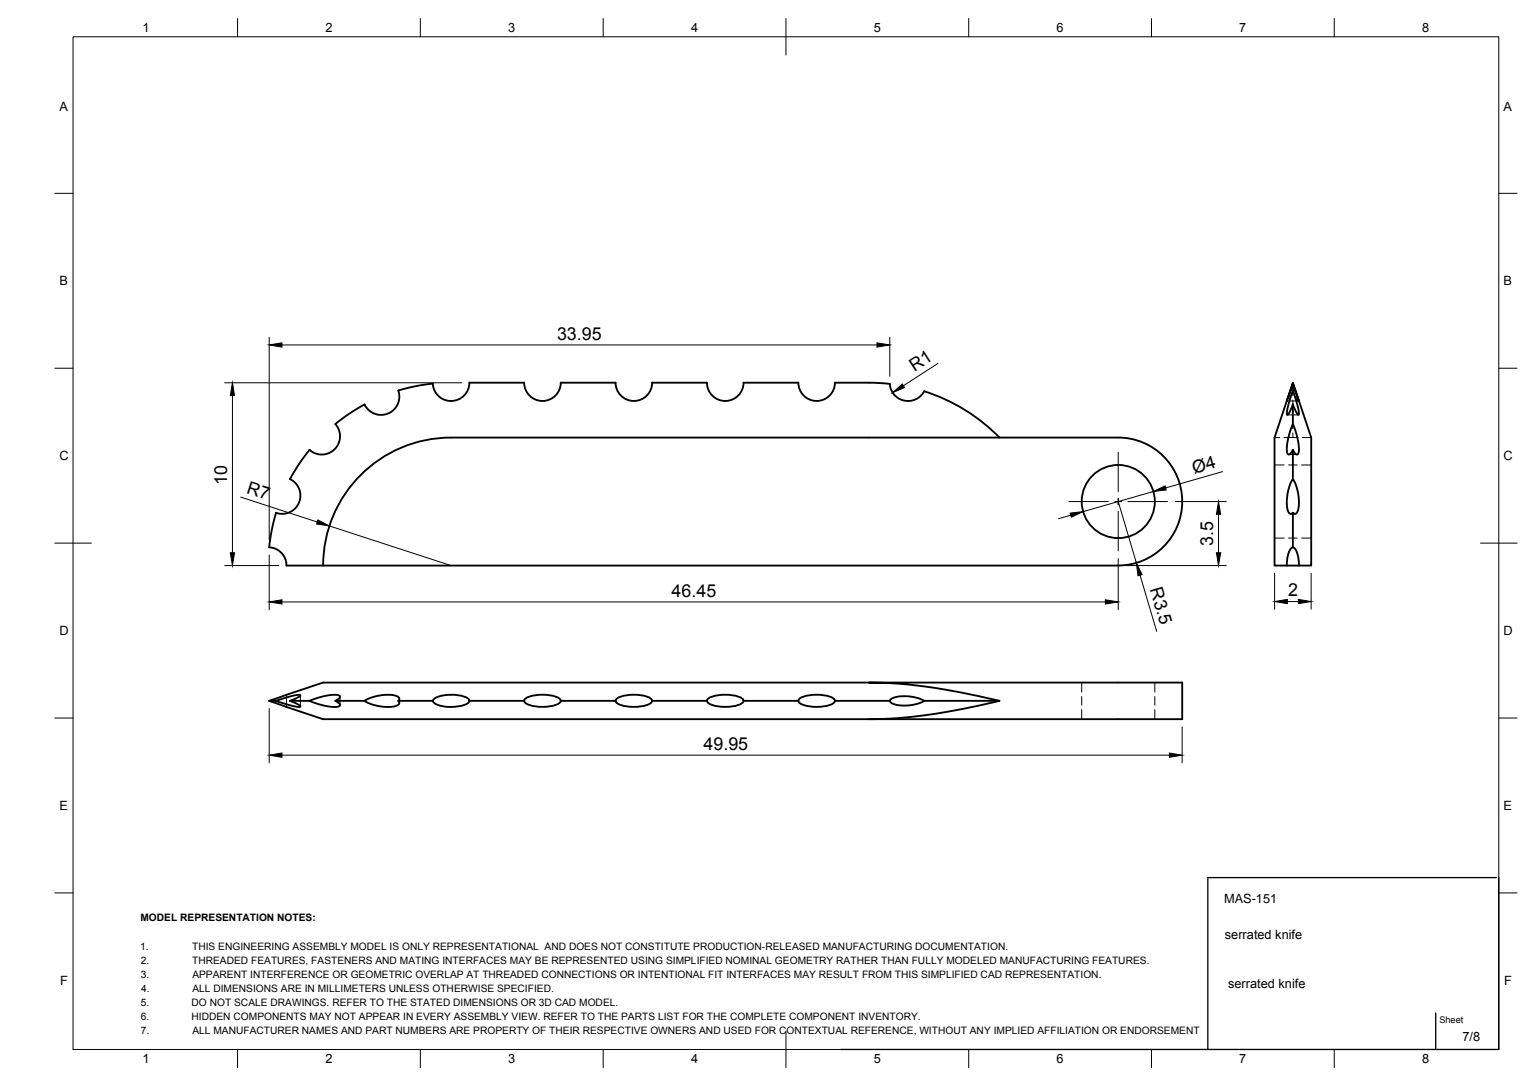
ISO-10303-21;
HEADER;
/* Generated by software containing ST-Developer
 * from STEP Tools, Inc. (www.steptools.com) 
 */

FILE_DESCRIPTION(
/* description */ ('STEP AP214'),
/* implementation_level */ '2;1');

FILE_NAME(
/* name */ 'serrated knife.step',
/* time_stamp */ '2026-11-04T19:14:12-08:00',
/* author */ (''),
/* organization */ (''),
/* preprocessor_version */ 'ST-DEVELOPER v20.2',
/* originating_system */ 'Autodesk Translation Framework v15.17.0.0',
/* authorisation */ '');

FILE_SCHEMA (('AUTOMOTIVE_DESIGN { 1 0 10303 214 3 1 1 }'));
ENDSEC;

DATA;
#10=MECHANICAL_DESIGN_GEOMETRIC_PRESENTATION_REPRESENTATION('',(#102),#5990);
#49=ELLIPSE('',#3546,1.05409255338808,0.99999999999868);
#50=ELLIPSE('',#3547,1.05409255338732,0.999999999998124);
#51=ELLIPSE('',#3549,1.05409255339022,1.00000000000065);
#52=ELLIPSE('',#3550,1.05409255338729,0.999999999997981);
#53=ELLIPSE('',#3552,1.05409255338844,0.99999999999902);
#54=ELLIPSE('',#3553,1.05409255338858,0.999999999999168);
#55=ELLIPSE('',#3555,1.05409255338794,0.999999999998691);
#56=ELLIPSE('',#3556,1.05409255338792,0.999999999998643);
#57=ELLIPSE('',#3558,1.05409255338783,0.999999999998475);
#58=ELLIPSE('',#3559,1.05409255338765,0.999999999998245);
#59=B_SPLINE_CURVE_WITH_KNOTS('',3,(#5264,#5265,#5266,#5267,#5268,#5269,
#5270,#5271,#5272,#5273,#5274,#5275,#5276,#5277,#5278,#5279,#5280,#5281),
 .UNSPECIFIED.,.F.,.F.,(4,2,2,2,2,2,2,2,4),(-0.601003528896593,-0.581975187755184,
-0.544665520692116,-0.509562261507989,-0.474459002323862,-0.439355743139737,
-0.404252483955611,-0.366942816892543,-0.347914475751133),.UNSPECIFIED.);
#60=B_SPLINE_CURVE_WITH_KNOTS('',3,(#5282,#5283,#5284,#5285,#5286,#5287,
#5288,#5289,#5290,#5291,#5292,#5293,#5294,#5295,#5296,#5297,#5298,#5299),
 .UNSPECIFIED.,.F.,.F.,(4,2,2,2,2,2,2,2,4),(-0.27137037906712,-0.252342037925712,
-0.215032370862644,-0.179929111678516,-0.144825852494388,-0.109722593310262,
-0.0746193341261349,-0.0373096670630674,-0.0182813259216579),
 .UNSPECIFIED.);
#61=B_SPLINE_CURVE_WITH_KNOTS('',3,(#5323,#5324,#5325,#5326,#5327,#5328,
#5329,#5330,#5331,#5332,#5333,#5334,#5335),.UNSPECIFIED.,.F.,.F.,(4,3,2,
2,2,4),(-0.00524378789543694,-6.24500451351651E-17,0.037252819941784,0.0745056398835681,
0.109553010570145,0.144600381256721),.UNSPECIFIED.);
#62=B_SPLINE_CURVE_WITH_KNOTS('',3,(#5340,#5341,#5342,#5343,#5344,#5345,
#5346,#5347,#5348,#5349,#5350,#5351,#5352),.UNSPECIFIED.,.F.,.F.,(4,2,2,
2,3,4),(-0.144600381256721,-0.109553010570144,-0.0745056398835681,-0.037252819941784,
5.55111512312578E-17,0.00524378789543793),.UNSPECIFIED.);
#63=B_SPLINE_CURVE_WITH_KNOTS('',3,(#5356,#5357,#5358,#5359,#5360,#5361,
#5362,#5363,#5364,#5365,#5366,#5367,#5368,#5369,#5370,#5371,#5372,#5373,
#5374,#5375,#5376,#5377,#5378),.UNSPECIFIED.,.F.,.F.,(4,3,2,2,2,2,2,2,2,
2,4),(-0.00524378789548939,0.,0.0372528199418273,0.0745056398836546,0.109553010570272,
0.144600381256889,0.179647751943506,0.214695122630123,0.25194794257195,
0.289200762513778,0.294444550409127),.UNSPECIFIED.);
#64=B_SPLINE_CURVE_WITH_KNOTS('',3,(#5379,#5380,#5381,#5382,#5383,#5384,
#5385,#5386,#5387,#5388,#5389,#5390,#5391,#5392,#5393,#5394,#5395,#5396,
#5397,#5398,#5399,#5400,#5401),.UNSPECIFIED.,.F.,.F.,(4,2,2,2,2,2,2,2,2,
3,4),(-0.294444550409266,-0.289200762513777,-0.25194794257195,-0.214695122630123,
-0.179647751943506,-0.144600381256889,-0.109553010570272,-0.0745056398836545,
-0.0372528199418273,0.,0.00524378789535096),.UNSPECIFIED.);
#65=B_SPLINE_CURVE_WITH_KNOTS('',3,(#5405,#5406,#5407,#5408,#5409,#5410,
#5411,#5412,#5413,#5414,#5415,#5416,#5417,#5418,#5419,#5420,#5421,#5422,
#5423,#5424,#5425,#5426,#5427),.UNSPECIFIED.,.F.,.F.,(4,3,2,2,2,2,2,2,2,
2,4),(-0.00524378789552401,0.,0.0372528199418277,0.0745056398836554,0.109553010570272,
0.144600381256889,0.179647751943506,0.214695122630123,0.25194794257195,
0.289200762513778,0.294444550409163),.UNSPECIFIED.);
#66=B_SPLINE_CURVE_WITH_KNOTS('',3,(#5428,#5429,#5430,#5431,#5432,#5433,
#5434,#5435,#5436,#5437,#5438,#5439,#5440,#5441,#5442,#5443,#5444,#5445,
#5446,#5447,#5448,#5449,#5450),.UNSPECIFIED.,.F.,.F.,(4,2,2,2,2,2,2,2,2,
3,4),(-0.294444550409303,-0.289200762513778,-0.25194794257195,-0.214695122630123,
-0.179647751943506,-0.144600381256889,-0.109553010570272,-0.0745056398836553,
-0.0372528199418277,0.,0.0052437878953856),.UNSPECIFIED.);
#67=B_SPLINE_CURVE_WITH_KNOTS('',3,(#5454,#5455,#5456,#5457,#5458,#5459,
#5460,#5461,#5462,#5463,#5464,#5465,#5466,#5467,#5468,#5469,#5470,#5471,
#5472,#5473,#5474,#5475,#5476),.UNSPECIFIED.,.F.,.F.,(4,3,2,2,2,2,2,2,2,
2,4),(-0.00524378789543961,0.,0.0372528199417981,0.0745056398835963,0.109553010570186,
0.144600381256775,0.179647751943365,0.214695122629955,0.251947942571753,
0.289200762513551,0.294444550408852),.UNSPECIFIED.);
#68=B_SPLINE_CURVE_WITH_KNOTS('',3,(#5477,#5478,#5479,#5480,#5481,#5482,
#5483,#5484,#5485,#5486,#5487,#5488,#5489,#5490,#5491,#5492,#5493,#5494,
#5495,#5496,#5497,#5498,#5499),.UNSPECIFIED.,.F.,.F.,(4,2,2,2,2,2,2,2,2,
3,4),(-0.294444550408994,-0.289200762513552,-0.251947942571754,-0.214695122629956,
-0.179647751943366,-0.144600381256776,-0.109553010570186,-0.0745056398835967,
-0.0372528199417983,0.,0.00524378789530167),.UNSPECIFIED.);
#69=B_SPLINE_CURVE_WITH_KNOTS('',3,(#5554,#5555,#5556,#5557,#5558,#5559,
#5560,#5561,#5562,#5563,#5564,#5565),.UNSPECIFIED.,.F.,.F.,(4,2,2,2,2,4),
(-0.294444550409229,-0.289200762513778,-0.251947942571951,-0.214695122630124,
-0.179647751943506,-0.144600381256889),.UNSPECIFIED.);
#70=B_SPLINE_CURVE_WITH_KNOTS('',3,(#5573,#5574,#5575,#5576,#5577,#5578,
#5579,#5580,#5581,#5582,#5583,#5584),.UNSPECIFIED.,.F.,.F.,(4,2,2,2,2,4),
(-0.474692173414376,-0.439644802727758,-0.404597432041141,-0.367344612099314,
-0.330091792157487,-0.324848004262036),.UNSPECIFIED.);
#77=CONICAL_SURFACE('',#3571,6.99999999999997,1.24904577239826);
#78=CONICAL_SURFACE('',#3575,6.99999999999997,1.24904577239826);
#79=CONICAL_SURFACE('',#3576,6.99999999999997,1.24904577239826);
#80=CONICAL_SURFACE('',#3582,6.99999999999997,1.24904577239826);
#83=(
BOUNDED_CURVE()
B_SPLINE_CURVE(2,(#5509,#5510,#5511),.UNSPECIFIED.,.F.,.F.)
B_SPLINE_CURVE_WITH_KNOTS((3,3),(1.46969384566992,2.45666783066588),
 .UNSPECIFIED.)
CURVE()
GEOMETRIC_REPRESENTATION_ITEM()
RATIONAL_B_SPLINE_CURVE((1.64285714285715,1.64285714285715,1.35294117647059))
REPRESENTATION_ITEM('')
);
#84=(
BOUNDED_CURVE()
B_SPLINE_CURVE(2,(#5512,#5513,#5514),.UNSPECIFIED.,.F.,.F.)
B_SPLINE_CURVE_WITH_KNOTS((3,3),(0.482719860673934,1.46969384566991),
 .UNSPECIFIED.)
CURVE()
GEOMETRIC_REPRESENTATION_ITEM()
RATIONAL_B_SPLINE_CURVE((1.35294117647058,1.64285714285714,1.64285714285714))
REPRESENTATION_ITEM('')
);
#88=SHAPE_REPRESENTATION_RELATIONSHIP('SRR','None',#6024,#95);
#95=ADVANCED_BREP_SHAPE_REPRESENTATION('',(#109),#5986);
#102=STYLED_ITEM('',(#6066),#109);
#109=MANIFOLD_SOLID_BREP('Body1',#3272);
#129=FACE_BOUND('',#557,.T.);
#130=FACE_BOUND('',#559,.T.);
#206=PLANE('',#3563);
#207=PLANE('',#3564);
#208=PLANE('',#3565);
#209=PLANE('',#3568);
#210=PLANE('',#3574);
#211=PLANE('',#3581);
#350=FACE_OUTER_BOUND('',#544,.T.);
#351=FACE_OUTER_BOUND('',#545,.T.);
#352=FACE_OUTER_BOUND('',#546,.T.);
#353=FACE_OUTER_BOUND('',#547,.T.);
#354=FACE_OUTER_BOUND('',#548,.T.);
#355=FACE_OUTER_BOUND('',#549,.T.);
#356=FACE_OUTER_BOUND('',#550,.T.);
#357=FACE_OUTER_BOUND('',#551,.T.);
#358=FACE_OUTER_BOUND('',#552,.T.);
#359=FACE_OUTER_BOUND('',#553,.T.);
#360=FACE_OUTER_BOUND('',#554,.T.);
#361=FACE_OUTER_BOUND('',#555,.T.);
#362=FACE_OUTER_BOUND('',#556,.T.);
#363=FACE_OUTER_BOUND('',#558,.T.);
#364=FACE_OUTER_BOUND('',#560,.T.);
#365=FACE_OUTER_BOUND('',#561,.T.);
#366=FACE_OUTER_BOUND('',#562,.T.);
#367=FACE_OUTER_BOUND('',#563,.T.);
#368=FACE_OUTER_BOUND('',#564,.T.);
#369=FACE_OUTER_BOUND('',#565,.T.);
#370=FACE_OUTER_BOUND('',#566,.T.);
#371=FACE_OUTER_BOUND('',#567,.T.);
#544=EDGE_LOOP('',(#2702,#2703,#2704,#2705));
#545=EDGE_LOOP('',(#2706,#2707));
#546=EDGE_LOOP('',(#2708,#2709));
#547=EDGE_LOOP('',(#2710,#2711));
#548=EDGE_LOOP('',(#2712,#2713));
#549=EDGE_LOOP('',(#2714,#2715));
#550=EDGE_LOOP('',(#2716,#2717,#2718,#2719));
#551=EDGE_LOOP('',(#2720,#2721));
#552=EDGE_LOOP('',(#2722,#2723));
#553=EDGE_LOOP('',(#2724,#2725));
#554=EDGE_LOOP('',(#2726,#2727,#2728,#2729,#2730));
#555=EDGE_LOOP('',(#2731,#2732,#2733,#2734,#2735,#2736));
#556=EDGE_LOOP('',(#2737,#2738,#2739,#2740,#2741));
#557=EDGE_LOOP('',(#2742));
#558=EDGE_LOOP('',(#2743,#2744,#2745,#2746,#2747));
#559=EDGE_LOOP('',(#2748));
#560=EDGE_LOOP('',(#2749,#2750,#2751,#2752,#2753));
#561=EDGE_LOOP('',(#2754,#2755,#2756,#2757,#2758,#2759,#2760,#2761,#2762,
#2763,#2764,#2765,#2766));
#562=EDGE_LOOP('',(#2767,#2768,#2769,#2770,#2771));
#563=EDGE_LOOP('',(#2772,#2773,#2774,#2775,#2776,#2777,#2778,#2779,#2780,
#2781,#2782,#2783));
#564=EDGE_LOOP('',(#2784,#2785,#2786,#2787,#2788,#2789,#2790,#2791,#2792,
#2793,#2794,#2795,#2796));
#565=EDGE_LOOP('',(#2797,#2798,#2799,#2800,#2801,#2802,#2803,#2804,#2805,
#2806,#2807,#2808));
#566=EDGE_LOOP('',(#2809,#2810,#2811));
#567=EDGE_LOOP('',(#2812,#2813,#2814,#2815));
#842=LINE('',#5259,#1145);
#843=LINE('',#5503,#1146);
#844=LINE('',#5505,#1147);
#845=LINE('',#5507,#1148);
#846=LINE('',#5518,#1149);
#847=LINE('',#5520,#1150);
#848=LINE('',#5522,#1151);
#849=LINE('',#5524,#1152);
#850=LINE('',#5526,#1153);
#851=LINE('',#5527,#1154);
#852=LINE('',#5531,#1155);
#853=LINE('',#5537,#1156);
#854=LINE('',#5541,#1157);
#855=LINE('',#5544,#1158);
#856=LINE('',#5545,#1159);
#857=LINE('',#5546,#1160);
#858=LINE('',#5547,#1161);
#859=LINE('',#5548,#1162);
#860=LINE('',#5549,#1163);
#861=LINE('',#5551,#1164);
#862=LINE('',#5571,#1165);
#1145=VECTOR('',#4283,2.);
#1146=VECTOR('',#4326,1000.);
#1147=VECTOR('',#4327,1000.);
#1148=VECTOR('',#4328,1000.);
#1149=VECTOR('',#4331,1000.);
#1150=VECTOR('',#4332,1000.);
#1151=VECTOR('',#4333,1000.);
#1152=VECTOR('',#4334,1000.);
#1153=VECTOR('',#4335,1000.);
#1154=VECTOR('',#4336,1000.);
#1155=VECTOR('',#4341,1000.);
#1156=VECTOR('',#4350,1000.);
#1157=VECTOR('',#4355,1000.);
#1158=VECTOR('',#4360,1000.);
#1159=VECTOR('',#4361,1000.);
#1160=VECTOR('',#4362,1000.);
#1161=VECTOR('',#4363,1000.);
#1162=VECTOR('',#4364,1000.);
#1163=VECTOR('',#4365,1000.);
#1164=VECTOR('',#4368,1000.);
#1165=VECTOR('',#4381,1000.);
#1302=CIRCLE('',#3542,2.);
#1303=CIRCLE('',#3543,2.);
#1304=CIRCLE('',#3566,3.5);
#1305=CIRCLE('',#3567,6.99999999999997);
#1306=CIRCLE('',#3569,3.5);
#1307=CIRCLE('',#3570,6.99999999999997);
#1308=CIRCLE('',#3572,10.);
#1309=CIRCLE('',#3573,10.);
#1310=CIRCLE('',#3577,10.);
#1311=CIRCLE('',#3578,10.);
#1312=CIRCLE('',#3579,10.);
#1313=CIRCLE('',#3580,10.);
#1548=VERTEX_POINT('',#5256);
#1549=VERTEX_POINT('',#5258);
#1550=VERTEX_POINT('',#5262);
#1551=VERTEX_POINT('',#5263);
#1552=VERTEX_POINT('',#5301);
#1553=VERTEX_POINT('',#5302);
#1554=VERTEX_POINT('',#5306);
#1555=VERTEX_POINT('',#5307);
#1556=VERTEX_POINT('',#5311);
#1557=VERTEX_POINT('',#5312);
#1558=VERTEX_POINT('',#5316);
#1559=VERTEX_POINT('',#5317);
#1560=VERTEX_POINT('',#5321);
#1561=VERTEX_POINT('',#5322);
#1562=VERTEX_POINT('',#5336);
#1563=VERTEX_POINT('',#5338);
#1564=VERTEX_POINT('',#5354);
#1565=VERTEX_POINT('',#5355);
#1566=VERTEX_POINT('',#5403);
#1567=VERTEX_POINT('',#5404);
#1568=VERTEX_POINT('',#5452);
#1569=VERTEX_POINT('',#5453);
#1570=VERTEX_POINT('',#5501);
#1571=VERTEX_POINT('',#5502);
#1572=VERTEX_POINT('',#5504);
#1573=VERTEX_POINT('',#5506);
#1574=VERTEX_POINT('',#5508);
#1575=VERTEX_POINT('',#5516);
#1576=VERTEX_POINT('',#5517);
#1577=VERTEX_POINT('',#5519);
#1578=VERTEX_POINT('',#5521);
#1579=VERTEX_POINT('',#5523);
#1580=VERTEX_POINT('',#5525);
#1581=VERTEX_POINT('',#5530);
#1582=VERTEX_POINT('',#5535);
#1583=VERTEX_POINT('',#5540);
#1584=VERTEX_POINT('',#5553);
#1947=EDGE_CURVE('',#1548,#1548,#1302,.T.);
#1948=EDGE_CURVE('',#1548,#1549,#842,.T.);
#1949=EDGE_CURVE('',#1549,#1549,#1303,.T.);
#1950=EDGE_CURVE('',#1550,#1551,#59,.T.);
#1951=EDGE_CURVE('',#1551,#1550,#60,.T.);
#1952=EDGE_CURVE('',#1552,#1553,#49,.T.);
#1953=EDGE_CURVE('',#1553,#1552,#50,.T.);
#1954=EDGE_CURVE('',#1554,#1555,#51,.T.);
#1955=EDGE_CURVE('',#1555,#1554,#52,.T.);
#1956=EDGE_CURVE('',#1556,#1557,#53,.T.);
#1957=EDGE_CURVE('',#1557,#1556,#54,.T.);
#1958=EDGE_CURVE('',#1558,#1559,#55,.T.);
#1959=EDGE_CURVE('',#1559,#1558,#56,.T.);
#1960=EDGE_CURVE('',#1560,#1561,#61,.T.);
#1961=EDGE_CURVE('',#1561,#1562,#57,.T.);
#1962=EDGE_CURVE('',#1562,#1563,#58,.T.);
#1963=EDGE_CURVE('',#1563,#1560,#62,.T.);
#1964=EDGE_CURVE('',#1564,#1565,#63,.T.);
#1965=EDGE_CURVE('',#1565,#1564,#64,.T.);
#1966=EDGE_CURVE('',#1566,#1567,#65,.T.);
#1967=EDGE_CURVE('',#1567,#1566,#66,.T.);
#1968=EDGE_CURVE('',#1568,#1569,#67,.T.);
#1969=EDGE_CURVE('',#1569,#1568,#68,.T.);
#1970=EDGE_CURVE('',#1570,#1571,#843,.T.);
#1971=EDGE_CURVE('',#1570,#1572,#844,.T.);
#1972=EDGE_CURVE('',#1572,#1573,#845,.T.);
#1973=EDGE_CURVE('',#1573,#1574,#83,.T.);
#1974=EDGE_CURVE('',#1574,#1571,#84,.T.);
#1975=EDGE_CURVE('',#1575,#1576,#846,.T.);
#1976=EDGE_CURVE('',#1575,#1577,#847,.T.);
#1977=EDGE_CURVE('',#1577,#1578,#848,.T.);
#1978=EDGE_CURVE('',#1578,#1579,#849,.T.);
#1979=EDGE_CURVE('',#1580,#1579,#850,.T.);
#1980=EDGE_CURVE('',#1580,#1576,#851,.T.);
#1981=EDGE_CURVE('',#1577,#1570,#1304,.T.);
#1982=EDGE_CURVE('',#1571,#1581,#852,.T.);
#1983=EDGE_CURVE('',#1581,#1578,#1305,.T.);
#1984=EDGE_CURVE('',#1572,#1575,#1306,.T.);
#1985=EDGE_CURVE('',#1576,#1582,#1307,.T.);
#1986=EDGE_CURVE('',#1582,#1573,#853,.T.);
#1987=EDGE_CURVE('',#1574,#1551,#1308,.T.);
#1988=EDGE_CURVE('',#1583,#1573,#854,.T.);
#1989=EDGE_CURVE('',#1550,#1583,#1309,.T.);
#1990=EDGE_CURVE('',#1583,#1553,#855,.T.);
#1991=EDGE_CURVE('',#1563,#1582,#856,.T.);
#1992=EDGE_CURVE('',#1558,#1562,#857,.T.);
#1993=EDGE_CURVE('',#1556,#1559,#858,.T.);
#1994=EDGE_CURVE('',#1554,#1557,#859,.T.);
#1995=EDGE_CURVE('',#1552,#1555,#860,.T.);
#1996=EDGE_CURVE('',#1571,#1583,#861,.T.);
#1997=EDGE_CURVE('',#1584,#1580,#69,.T.);
#1998=EDGE_CURVE('',#1564,#1584,#1310,.T.);
#1999=EDGE_CURVE('',#1566,#1565,#1311,.T.);
#2000=EDGE_CURVE('',#1568,#1567,#1312,.T.);
#2001=EDGE_CURVE('',#1560,#1569,#1313,.T.);
#2002=EDGE_CURVE('',#1581,#1561,#862,.T.);
#2003=EDGE_CURVE('',#1579,#1584,#70,.T.);
#2702=ORIENTED_EDGE('',*,*,#1947,.F.);
#2703=ORIENTED_EDGE('',*,*,#1948,.T.);
#2704=ORIENTED_EDGE('',*,*,#1949,.F.);
#2705=ORIENTED_EDGE('',*,*,#1948,.F.);
#2706=ORIENTED_EDGE('',*,*,#1950,.T.);
#2707=ORIENTED_EDGE('',*,*,#1951,.T.);
#2708=ORIENTED_EDGE('',*,*,#1952,.T.);
#2709=ORIENTED_EDGE('',*,*,#1953,.T.);
#2710=ORIENTED_EDGE('',*,*,#1954,.T.);
#2711=ORIENTED_EDGE('',*,*,#1955,.T.);
#2712=ORIENTED_EDGE('',*,*,#1956,.T.);
#2713=ORIENTED_EDGE('',*,*,#1957,.T.);
#2714=ORIENTED_EDGE('',*,*,#1958,.T.);
#2715=ORIENTED_EDGE('',*,*,#1959,.T.);
#2716=ORIENTED_EDGE('',*,*,#1960,.T.);
#2717=ORIENTED_EDGE('',*,*,#1961,.T.);
#2718=ORIENTED_EDGE('',*,*,#1962,.T.);
#2719=ORIENTED_EDGE('',*,*,#1963,.T.);
#2720=ORIENTED_EDGE('',*,*,#1964,.T.);
#2721=ORIENTED_EDGE('',*,*,#1965,.T.);
#2722=ORIENTED_EDGE('',*,*,#1966,.T.);
#2723=ORIENTED_EDGE('',*,*,#1967,.T.);
#2724=ORIENTED_EDGE('',*,*,#1968,.T.);
#2725=ORIENTED_EDGE('',*,*,#1969,.T.);
#2726=ORIENTED_EDGE('',*,*,#1970,.F.);
#2727=ORIENTED_EDGE('',*,*,#1971,.T.);
#2728=ORIENTED_EDGE('',*,*,#1972,.T.);
#2729=ORIENTED_EDGE('',*,*,#1973,.T.);
#2730=ORIENTED_EDGE('',*,*,#1974,.T.);
#2731=ORIENTED_EDGE('',*,*,#1975,.F.);
#2732=ORIENTED_EDGE('',*,*,#1976,.T.);
#2733=ORIENTED_EDGE('',*,*,#1977,.T.);
#2734=ORIENTED_EDGE('',*,*,#1978,.T.);
#2735=ORIENTED_EDGE('',*,*,#1979,.F.);
#2736=ORIENTED_EDGE('',*,*,#1980,.T.);
#2737=ORIENTED_EDGE('',*,*,#1977,.F.);
#2738=ORIENTED_EDGE('',*,*,#1981,.T.);
#2739=ORIENTED_EDGE('',*,*,#1970,.T.);
#2740=ORIENTED_EDGE('',*,*,#1982,.T.);
#2741=ORIENTED_EDGE('',*,*,#1983,.T.);
#2742=ORIENTED_EDGE('',*,*,#1947,.T.);
#2743=ORIENTED_EDGE('',*,*,#1984,.T.);
#2744=ORIENTED_EDGE('',*,*,#1975,.T.);
#2745=ORIENTED_EDGE('',*,*,#1985,.T.);
#2746=ORIENTED_EDGE('',*,*,#1986,.T.);
#2747=ORIENTED_EDGE('',*,*,#1972,.F.);
#2748=ORIENTED_EDGE('',*,*,#1949,.T.);
#2749=ORIENTED_EDGE('',*,*,#1951,.F.);
#2750=ORIENTED_EDGE('',*,*,#1987,.F.);
#2751=ORIENTED_EDGE('',*,*,#1973,.F.);
#2752=ORIENTED_EDGE('',*,*,#1988,.F.);
#2753=ORIENTED_EDGE('',*,*,#1989,.F.);
#2754=ORIENTED_EDGE('',*,*,#1953,.F.);
#2755=ORIENTED_EDGE('',*,*,#1990,.F.);
#2756=ORIENTED_EDGE('',*,*,#1988,.T.);
#2757=ORIENTED_EDGE('',*,*,#1986,.F.);
#2758=ORIENTED_EDGE('',*,*,#1991,.F.);
#2759=ORIENTED_EDGE('',*,*,#1962,.F.);
#2760=ORIENTED_EDGE('',*,*,#1992,.F.);
#2761=ORIENTED_EDGE('',*,*,#1959,.F.);
#2762=ORIENTED_EDGE('',*,*,#1993,.F.);
#2763=ORIENTED_EDGE('',*,*,#1957,.F.);
#2764=ORIENTED_EDGE('',*,*,#1994,.F.);
#2765=ORIENTED_EDGE('',*,*,#1955,.F.);
#2766=ORIENTED_EDGE('',*,*,#1995,.F.);
#2767=ORIENTED_EDGE('',*,*,#1950,.F.);
#2768=ORIENTED_EDGE('',*,*,#1989,.T.);
#2769=ORIENTED_EDGE('',*,*,#1996,.F.);
#2770=ORIENTED_EDGE('',*,*,#1974,.F.);
#2771=ORIENTED_EDGE('',*,*,#1987,.T.);
#2772=ORIENTED_EDGE('',*,*,#1997,.F.);
#2773=ORIENTED_EDGE('',*,*,#1998,.F.);
#2774=ORIENTED_EDGE('',*,*,#1965,.F.);
#2775=ORIENTED_EDGE('',*,*,#1999,.F.);
#2776=ORIENTED_EDGE('',*,*,#1967,.F.);
#2777=ORIENTED_EDGE('',*,*,#2000,.F.);
#2778=ORIENTED_EDGE('',*,*,#1969,.F.);
#2779=ORIENTED_EDGE('',*,*,#2001,.F.);
#2780=ORIENTED_EDGE('',*,*,#1963,.F.);
#2781=ORIENTED_EDGE('',*,*,#1991,.T.);
#2782=ORIENTED_EDGE('',*,*,#1985,.F.);
#2783=ORIENTED_EDGE('',*,*,#1980,.F.);
#2784=ORIENTED_EDGE('',*,*,#1952,.F.);
#2785=ORIENTED_EDGE('',*,*,#1995,.T.);
#2786=ORIENTED_EDGE('',*,*,#1954,.F.);
#2787=ORIENTED_EDGE('',*,*,#1994,.T.);
#2788=ORIENTED_EDGE('',*,*,#1956,.F.);
#2789=ORIENTED_EDGE('',*,*,#1993,.T.);
#2790=ORIENTED_EDGE('',*,*,#1958,.F.);
#2791=ORIENTED_EDGE('',*,*,#1992,.T.);
#2792=ORIENTED_EDGE('',*,*,#1961,.F.);
#2793=ORIENTED_EDGE('',*,*,#2002,.F.);
#2794=ORIENTED_EDGE('',*,*,#1982,.F.);
#2795=ORIENTED_EDGE('',*,*,#1996,.T.);
#2796=ORIENTED_EDGE('',*,*,#1990,.T.);
#2797=ORIENTED_EDGE('',*,*,#2003,.F.);
#2798=ORIENTED_EDGE('',*,*,#1978,.F.);
#2799=ORIENTED_EDGE('',*,*,#1983,.F.);
#2800=ORIENTED_EDGE('',*,*,#2002,.T.);
#2801=ORIENTED_EDGE('',*,*,#1960,.F.);
#2802=ORIENTED_EDGE('',*,*,#2001,.T.);
#2803=ORIENTED_EDGE('',*,*,#1968,.F.);
#2804=ORIENTED_EDGE('',*,*,#2000,.T.);
#2805=ORIENTED_EDGE('',*,*,#1966,.F.);
#2806=ORIENTED_EDGE('',*,*,#1999,.T.);
#2807=ORIENTED_EDGE('',*,*,#1964,.F.);
#2808=ORIENTED_EDGE('',*,*,#1998,.T.);
#2809=ORIENTED_EDGE('',*,*,#1979,.T.);
#2810=ORIENTED_EDGE('',*,*,#2003,.T.);
#2811=ORIENTED_EDGE('',*,*,#1997,.T.);
#2812=ORIENTED_EDGE('',*,*,#1971,.F.);
#2813=ORIENTED_EDGE('',*,*,#1981,.F.);
#2814=ORIENTED_EDGE('',*,*,#1976,.F.);
#2815=ORIENTED_EDGE('',*,*,#1984,.F.);
#3063=CYLINDRICAL_SURFACE('',#3541,2.);
#3064=CYLINDRICAL_SURFACE('',#3544,0.999999999998776);
#3065=CYLINDRICAL_SURFACE('',#3545,0.999999999998766);
#3066=CYLINDRICAL_SURFACE('',#3548,0.999999999998766);
#3067=CYLINDRICAL_SURFACE('',#3551,0.999999999998766);
#3068=CYLINDRICAL_SURFACE('',#3554,0.999999999998766);
#3069=CYLINDRICAL_SURFACE('',#3557,0.999999999998766);
#3070=CYLINDRICAL_SURFACE('',#3560,1.);
#3071=CYLINDRICAL_SURFACE('',#3561,1.00000000000001);
#3072=CYLINDRICAL_SURFACE('',#3562,0.999999999999161);
#3073=CYLINDRICAL_SURFACE('',#3583,1.);
#3074=CYLINDRICAL_SURFACE('',#3584,3.5);
#3199=ADVANCED_FACE('',(#350),#3063,.F.);
#3200=ADVANCED_FACE('',(#351),#3064,.F.);
#3201=ADVANCED_FACE('',(#352),#3065,.F.);
#3202=ADVANCED_FACE('',(#353),#3066,.F.);
#3203=ADVANCED_FACE('',(#354),#3067,.F.);
#3204=ADVANCED_FACE('',(#355),#3068,.F.);
#3205=ADVANCED_FACE('',(#356),#3069,.F.);
#3206=ADVANCED_FACE('',(#357),#3070,.F.);
#3207=ADVANCED_FACE('',(#358),#3071,.F.);
#3208=ADVANCED_FACE('',(#359),#3072,.F.);
#3209=ADVANCED_FACE('',(#360),#206,.F.);
#3210=ADVANCED_FACE('',(#361),#207,.T.);
#3211=ADVANCED_FACE('',(#362,#129),#208,.T.);
#3212=ADVANCED_FACE('',(#363,#130),#209,.F.);
#3213=ADVANCED_FACE('',(#364),#77,.T.);
#3214=ADVANCED_FACE('',(#365),#210,.T.);
#3215=ADVANCED_FACE('',(#366),#78,.T.);
#3216=ADVANCED_FACE('',(#367),#79,.T.);
#3217=ADVANCED_FACE('',(#368),#211,.F.);
#3218=ADVANCED_FACE('',(#369),#80,.T.);
#3219=ADVANCED_FACE('',(#370),#3073,.F.);
#3220=ADVANCED_FACE('',(#371),#3074,.T.);
#3272=CLOSED_SHELL('',(#3199,#3200,#3201,#3202,#3203,#3204,#3205,#3206,
#3207,#3208,#3209,#3210,#3211,#3212,#3213,#3214,#3215,#3216,#3217,#3218,
#3219,#3220));
#3540=AXIS2_PLACEMENT_3D('',#5254,#4277,#4278);
#3541=AXIS2_PLACEMENT_3D('',#5255,#4279,#4280);
#3542=AXIS2_PLACEMENT_3D('',#5257,#4281,#4282);
#3543=AXIS2_PLACEMENT_3D('',#5260,#4284,#4285);
#3544=AXIS2_PLACEMENT_3D('',#5261,#4286,#4287);
#3545=AXIS2_PLACEMENT_3D('',#5300,#4288,#4289);
#3546=AXIS2_PLACEMENT_3D('',#5303,#4290,#4291);
#3547=AXIS2_PLACEMENT_3D('',#5304,#4292,#4293);
#3548=AXIS2_PLACEMENT_3D('',#5305,#4294,#4295);
#3549=AXIS2_PLACEMENT_3D('',#5308,#4296,#4297);
#3550=AXIS2_PLACEMENT_3D('',#5309,#4298,#4299);
#3551=AXIS2_PLACEMENT_3D('',#5310,#4300,#4301);
#3552=AXIS2_PLACEMENT_3D('',#5313,#4302,#4303);
#3553=AXIS2_PLACEMENT_3D('',#5314,#4304,#4305);
#3554=AXIS2_PLACEMENT_3D('',#5315,#4306,#4307);
#3555=AXIS2_PLACEMENT_3D('',#5318,#4308,#4309);
#3556=AXIS2_PLACEMENT_3D('',#5319,#4310,#4311);
#3557=AXIS2_PLACEMENT_3D('',#5320,#4312,#4313);
#3558=AXIS2_PLACEMENT_3D('',#5337,#4314,#4315);
#3559=AXIS2_PLACEMENT_3D('',#5339,#4316,#4317);
#3560=AXIS2_PLACEMENT_3D('',#5353,#4318,#4319);
#3561=AXIS2_PLACEMENT_3D('',#5402,#4320,#4321);
#3562=AXIS2_PLACEMENT_3D('',#5451,#4322,#4323);
#3563=AXIS2_PLACEMENT_3D('',#5500,#4324,#4325);
#3564=AXIS2_PLACEMENT_3D('',#5515,#4329,#4330);
#3565=AXIS2_PLACEMENT_3D('',#5528,#4337,#4338);
#3566=AXIS2_PLACEMENT_3D('',#5529,#4339,#4340);
#3567=AXIS2_PLACEMENT_3D('',#5532,#4342,#4343);
#3568=AXIS2_PLACEMENT_3D('',#5533,#4344,#4345);
#3569=AXIS2_PLACEMENT_3D('',#5534,#4346,#4347);
#3570=AXIS2_PLACEMENT_3D('',#5536,#4348,#4349);
#3571=AXIS2_PLACEMENT_3D('',#5538,#4351,#4352);
#3572=AXIS2_PLACEMENT_3D('',#5539,#4353,#4354);
#3573=AXIS2_PLACEMENT_3D('',#5542,#4356,#4357);
#3574=AXIS2_PLACEMENT_3D('',#5543,#4358,#4359);
#3575=AXIS2_PLACEMENT_3D('',#5550,#4366,#4367);
#3576=AXIS2_PLACEMENT_3D('',#5552,#4369,#4370);
#3577=AXIS2_PLACEMENT_3D('',#5566,#4371,#4372);
#3578=AXIS2_PLACEMENT_3D('',#5567,#4373,#4374);
#3579=AXIS2_PLACEMENT_3D('',#5568,#4375,#4376);
#3580=AXIS2_PLACEMENT_3D('',#5569,#4377,#4378);
#3581=AXIS2_PLACEMENT_3D('',#5570,#4379,#4380);
#3582=AXIS2_PLACEMENT_3D('',#5572,#4382,#4383);
#3583=AXIS2_PLACEMENT_3D('',#5585,#4384,#4385);
#3584=AXIS2_PLACEMENT_3D('',#5586,#4386,#4387);
#4277=DIRECTION('axis',(0.,0.,1.));
#4278=DIRECTION('refdir',(1.,0.,0.));
#4279=DIRECTION('center_axis',(4.4406667760173E-16,2.77555573237168E-17,
1.));
#4280=DIRECTION('ref_axis',(1.,-2.43623723452952E-32,-4.4406667760173E-16));
#4281=DIRECTION('center_axis',(4.4406667760173E-16,2.77555573237168E-17,
1.));
#4282=DIRECTION('ref_axis',(1.,-2.43623723452952E-32,-4.4406667760173E-16));
#4283=DIRECTION('',(4.4406667760173E-16,2.77555573237168E-17,1.));
#4284=DIRECTION('center_axis',(-4.4406667760173E-16,-2.77555573237168E-17,
-1.));
#4285=DIRECTION('ref_axis',(-1.,2.46506362514545E-32,4.4406667760173E-16));
#4286=DIRECTION('center_axis',(4.4406667760173E-16,2.77555573237168E-17,
1.));
#4287=DIRECTION('ref_axis',(1.,-2.43623723453099E-32,-4.4406667760173E-16));
#4288=DIRECTION('center_axis',(4.4406667760173E-16,2.77555573237168E-17,
1.));
#4289=DIRECTION('ref_axis',(1.,-2.436237234531E-32,-4.4406667760173E-16));
#4290=DIRECTION('center_axis',(-0.316227766016829,3.0018299425529E-15,-0.948683298050517));
#4291=DIRECTION('ref_axis',(0.948683298050517,-9.96757165847559E-13,-0.316227766016829));
#4292=DIRECTION('center_axis',(-0.316227766016834,-7.50457485638231E-16,
0.948683298050515));
#4293=DIRECTION('ref_axis',(0.948683298050515,-6.16711447781422E-12,0.316227766016834));
#4294=DIRECTION('center_axis',(4.4406667760173E-16,2.77555573237168E-17,
1.));
#4295=DIRECTION('ref_axis',(1.,-2.436237234531E-32,-4.4406667760173E-16));
#4296=DIRECTION('center_axis',(-0.316227766016829,3.11728494034299E-15,
-0.948683298050517));
#4297=DIRECTION('ref_axis',(0.948683298050517,1.56058638540273E-11,-0.316227766016829));
#4298=DIRECTION('center_axis',(-0.316227766016834,-7.50457485638232E-16,
0.948683298050515));
#4299=DIRECTION('ref_axis',(0.948683298050515,-6.59186276791152E-12,0.316227766016834));
#4300=DIRECTION('center_axis',(4.4406667760173E-16,2.77555573237168E-17,
1.));
#4301=DIRECTION('ref_axis',(1.,-2.436237234531E-32,-4.4406667760173E-16));
#4302=DIRECTION('center_axis',(-0.31622776601683,2.77091994697168E-15,-0.948683298050517));
#4303=DIRECTION('ref_axis',(0.948683298050517,2.37176708321596E-12,-0.31622776601683));
#4304=DIRECTION('center_axis',(-0.316227766016833,3.4636499337146E-16,0.948683298050515));
#4305=DIRECTION('ref_axis',(0.948683298050515,3.44351511508786E-12,0.316227766016833));
#4306=DIRECTION('center_axis',(4.4406667760173E-16,2.77555573237168E-17,
1.));
#4307=DIRECTION('ref_axis',(1.,-2.436237234531E-32,-4.4406667760173E-16));
#4308=DIRECTION('center_axis',(-0.31622776601683,2.77091994697168E-15,-0.948683298050517));
#4309=DIRECTION('ref_axis',(0.948683298050517,-7.95145482367482E-13,-0.31622776601683));
#4310=DIRECTION('center_axis',(-0.316227766016833,3.4636499337146E-16,0.948683298050515));
#4311=DIRECTION('ref_axis',(0.948683298050515,-1.06976938896506E-12,0.316227766016833));
#4312=DIRECTION('center_axis',(4.4406667760173E-16,2.77555573237168E-17,
1.));
#4313=DIRECTION('ref_axis',(1.,-2.436237234531E-32,-4.4406667760173E-16));
#4314=DIRECTION('center_axis',(-0.316227766016832,-2.02046246133356E-16,
-0.948683298050516));
#4315=DIRECTION('ref_axis',(0.948683298050516,2.39882550987045E-12,-0.316227766016832));
#4316=DIRECTION('center_axis',(-0.316227766016834,1.15454997790497E-16,
0.948683298050515));
#4317=DIRECTION('ref_axis',(0.948683298050515,4.35170492897026E-12,0.316227766016834));
#4318=DIRECTION('center_axis',(4.4406667760173E-16,2.77555573237168E-17,
1.));
#4319=DIRECTION('ref_axis',(1.,-2.43623723452951E-32,-4.4406667760173E-16));
#4320=DIRECTION('center_axis',(4.4406667760173E-16,2.77555573237168E-17,
1.));
#4321=DIRECTION('ref_axis',(1.,-2.43623723452951E-32,-4.4406667760173E-16));
#4322=DIRECTION('center_axis',(4.4406667760173E-16,2.77555573237168E-17,
1.));
#4323=DIRECTION('ref_axis',(1.,-2.43623723453053E-32,-4.4406667760173E-16));
#4324=DIRECTION('center_axis',(1.,6.93889390390723E-17,-4.4406667760173E-16));
#4325=DIRECTION('ref_axis',(-4.4406667760173E-16,-2.77555573237168E-17,
-1.));
#4326=DIRECTION('',(6.93889390390723E-17,1.,2.77555573237168E-17));
#4327=DIRECTION('',(4.4406667760173E-16,2.77555573237168E-17,1.));
#4328=DIRECTION('',(6.93889390390723E-17,1.,2.77555573237168E-17));
#4329=DIRECTION('center_axis',(1.,6.93889390390723E-17,-4.4406667760173E-16));
#4330=DIRECTION('ref_axis',(-4.4406667760173E-16,-2.77555573237168E-17,
-1.));
#4331=DIRECTION('',(6.93889390390723E-17,1.,2.77555573237168E-17));
#4332=DIRECTION('',(-4.4406667760173E-16,-2.77555573237168E-17,-1.));
#4333=DIRECTION('',(6.93889390390723E-17,1.,2.77555573237168E-17));
#4334=DIRECTION('',(2.06254340956326E-16,0.948683298050515,0.316227766016835));
#4335=DIRECTION('',(-4.4406667760173E-16,-2.77555573237168E-17,-1.));
#4336=DIRECTION('',(7.45980858847001E-17,-0.948683298050515,0.316227766016835));
#4337=DIRECTION('center_axis',(4.4406667760173E-16,-2.77555573237167E-17,
-1.));
#4338=DIRECTION('ref_axis',(-1.,-6.93889390390723E-17,-4.4406667760173E-16));
#4339=DIRECTION('center_axis',(-4.4406667760173E-16,-2.77555573237168E-17,
-1.));
#4340=DIRECTION('ref_axis',(-1.,2.60819515195191E-32,4.4406667760173E-16));
#4341=DIRECTION('',(6.93889390390723E-17,1.,2.77555573237168E-17));
#4342=DIRECTION('center_axis',(-4.4406667760173E-16,-2.77555573237168E-17,
-1.));
#4343=DIRECTION('ref_axis',(-1.,2.43623723452952E-32,4.4406667760173E-16));
#4344=DIRECTION('center_axis',(4.4406667760173E-16,-2.77555573237167E-17,
-1.));
#4345=DIRECTION('ref_axis',(-1.,-6.93889390390723E-17,-4.4406667760173E-16));
#4346=DIRECTION('center_axis',(4.4406667760173E-16,2.77555573237168E-17,
1.));
#4347=DIRECTION('ref_axis',(-1.,2.46506362514546E-32,4.4406667760173E-16));
#4348=DIRECTION('center_axis',(4.4406667760173E-16,2.77555573237168E-17,
1.));
#4349=DIRECTION('ref_axis',(-1.,2.46506362514546E-32,4.4406667760173E-16));
#4350=DIRECTION('',(-6.93889390390723E-17,-1.,-2.77555573237168E-17));
#4351=DIRECTION('center_axis',(-4.4406667760173E-16,-2.77555573237168E-17,
-1.));
#4352=DIRECTION('ref_axis',(-1.,2.46506362514546E-32,4.4406667760173E-16));
#4353=DIRECTION('center_axis',(-4.4406667760173E-16,-2.77555573237168E-17,
-1.));
#4354=DIRECTION('ref_axis',(-1.,2.43623723452952E-32,4.4406667760173E-16));
#4355=DIRECTION('',(0.948683298050515,7.46052054228444E-17,0.316227766016835));
#4356=DIRECTION('center_axis',(-4.4406667760173E-16,-2.77555573237168E-17,
-1.));
#4357=DIRECTION('ref_axis',(-1.,2.43623723452952E-32,4.4406667760173E-16));
#4358=DIRECTION('center_axis',(-0.316227766016835,-4.38852448248957E-18,
0.948683298050515));
#4359=DIRECTION('ref_axis',(-6.93889390390723E-17,-1.,-2.77555573237168E-17));
#4360=DIRECTION('',(6.93889390390723E-17,1.,2.77555573237168E-17));
#4361=DIRECTION('',(0.948683298050515,7.46052054228444E-17,0.316227766016835));
#4362=DIRECTION('',(6.93889390390723E-17,1.,2.77555573237168E-17));
#4363=DIRECTION('',(6.93889390390723E-17,1.,2.77555573237168E-17));
#4364=DIRECTION('',(6.93889390390723E-17,1.,2.77555573237168E-17));
#4365=DIRECTION('',(6.93889390390723E-17,1.,2.77555573237168E-17));
#4366=DIRECTION('center_axis',(4.4406667760173E-16,2.77555573237168E-17,
1.));
#4367=DIRECTION('ref_axis',(1.,-2.43623723452952E-32,-4.4406667760173E-16));
#4368=DIRECTION('',(-0.948683298050515,-5.7051049648782E-17,0.316227766016835));
#4369=DIRECTION('center_axis',(-4.4406667760173E-16,-2.77555573237168E-17,
-1.));
#4370=DIRECTION('ref_axis',(-1.,2.46506362514546E-32,4.4406667760173E-16));
#4371=DIRECTION('center_axis',(-4.4406667760173E-16,-2.77555573237168E-17,
-1.));
#4372=DIRECTION('ref_axis',(-1.,2.43623723452952E-32,4.4406667760173E-16));
#4373=DIRECTION('center_axis',(-4.4406667760173E-16,-2.77555573237168E-17,
-1.));
#4374=DIRECTION('ref_axis',(-1.,2.43623723452952E-32,4.4406667760173E-16));
#4375=DIRECTION('center_axis',(-4.4406667760173E-16,-2.77555573237168E-17,
-1.));
#4376=DIRECTION('ref_axis',(-1.,2.43623723452952E-32,4.4406667760173E-16));
#4377=DIRECTION('center_axis',(-4.4406667760173E-16,-2.77555573237168E-17,
-1.));
#4378=DIRECTION('ref_axis',(-1.,2.43623723452952E-32,4.4406667760173E-16));
#4379=DIRECTION('center_axis',(0.316227766016835,-4.8273942839698E-17,0.948683298050515));
#4380=DIRECTION('ref_axis',(-6.93889390390723E-17,-1.,-2.77555573237168E-17));
#4381=DIRECTION('',(-0.948683298050515,-5.7051049648782E-17,0.316227766016835));
#4382=DIRECTION('center_axis',(4.4406667760173E-16,2.77555573237168E-17,
1.));
#4383=DIRECTION('ref_axis',(1.,-2.43623723452952E-32,-4.4406667760173E-16));
#4384=DIRECTION('center_axis',(4.4406667760173E-16,2.77555573237168E-17,
1.));
#4385=DIRECTION('ref_axis',(1.,-2.43623723452951E-32,-4.4406667760173E-16));
#4386=DIRECTION('center_axis',(4.4406667760173E-16,2.77555573237168E-17,
1.));
#4387=DIRECTION('ref_axis',(1.,-2.60819515195191E-32,-4.4406667760173E-16));
#5254=CARTESIAN_POINT('',(0.,0.,0.));
#5255=CARTESIAN_POINT('Origin',(-16.,-116.5,-2.00000000000001));
#5256=CARTESIAN_POINT('',(-18.,-116.5,-2.00000000000001));
#5257=CARTESIAN_POINT('Origin',(-16.,-116.5,-2.00000000000001));
#5258=CARTESIAN_POINT('',(-18.,-116.5,-1.30451205393456E-14));
#5259=CARTESIAN_POINT('',(-18.,-116.5,-2.00000000000001));
#5260=CARTESIAN_POINT('Origin',(-16.,-116.5,-1.38777878078145E-14));
#5261=CARTESIAN_POINT('Origin',(-22.5,-105.,-1.50000000000001));
#5262=CARTESIAN_POINT('',(-22.4343957334051,-104.002154280361,-1.00000000000001));
#5263=CARTESIAN_POINT('',(-22.0315240935613,-105.883476273074,-1.00000000000001));
#5264=CARTESIAN_POINT('Ctrl Pts',(-22.4343957334051,-104.002154280361,-1.00000000000001));
#5265=CARTESIAN_POINT('Ctrl Pts',(-22.3711029895888,-104.006315518874,-1.02080054812375));
#5266=CARTESIAN_POINT('Ctrl Pts',(-22.3070770846659,-104.016655879379,-1.04160380896525));
#5267=CARTESIAN_POINT('Ctrl Pts',(-22.1218994092456,-104.065586327466,-1.10093418649023));
#5268=CARTESIAN_POINT('Ctrl Pts',(-22.0050091877668,-104.122719505682,-1.13722283104251));
#5269=CARTESIAN_POINT('Ctrl Pts',(-21.8158438636493,-104.261835149209,-1.19313252973015));
#5270=CARTESIAN_POINT('Ctrl Pts',(-21.7287811554342,-104.351555835029,-1.21730844885347));
#5271=CARTESIAN_POINT('Ctrl Pts',(-21.5941724070256,-104.558712433615,-1.24965683324256));
#5272=CARTESIAN_POINT('Ctrl Pts',(-21.5466705229745,-104.676187630697,-1.25776140553084));
#5273=CARTESIAN_POINT('Ctrl Pts',(-21.4976674225048,-104.905021337286,-1.25776140553084));
#5274=CARTESIAN_POINT('Ctrl Pts',(-21.4928968258581,-105.031647133732,-1.24965683324256));
#5275=CARTESIAN_POINT('Ctrl Pts',(-21.5308692848446,-105.275760762692,-1.21730844885347));
#5276=CARTESIAN_POINT('Ctrl Pts',(-21.5735559693207,-105.393266352322,-1.19313252973015));
#5277=CARTESIAN_POINT('Ctrl Pts',(-21.6891640143735,-105.597647031549,-1.13722283104251));
#5278=CARTESIAN_POINT('Ctrl Pts',(-21.7724073571378,-105.697637380163,-1.10093418649023));
#5279=CARTESIAN_POINT('Ctrl Pts',(-21.9213088988862,-105.818108501553,-1.04160380896526));
#5280=CARTESIAN_POINT('Ctrl Pts',(-21.975485733804,-105.8537611328,-1.02080054812375));
#5281=CARTESIAN_POINT('Ctrl Pts',(-22.0315240935613,-105.883476273074,-1.00000000000001));
#5282=CARTESIAN_POINT('Ctrl Pts',(-22.0315240935613,-105.883476273074,-1.00000000000001));
#5283=CARTESIAN_POINT('Ctrl Pts',(-21.975485733804,-105.8537611328,-0.979199451876273));
#5284=CARTESIAN_POINT('Ctrl Pts',(-21.9213088988862,-105.818108501553,-0.958396191034767));
#5285=CARTESIAN_POINT('Ctrl Pts',(-21.7724073571378,-105.697637380163,-0.899065813509789));
#5286=CARTESIAN_POINT('Ctrl Pts',(-21.6891640143735,-105.597647031549,-0.862777168957508));
#5287=CARTESIAN_POINT('Ctrl Pts',(-21.5735559693207,-105.393266352322,-0.806867470269865));
#5288=CARTESIAN_POINT('Ctrl Pts',(-21.5308692848446,-105.275760762692,-0.782691551146544));
#5289=CARTESIAN_POINT('Ctrl Pts',(-21.4928968258581,-105.031647133732,-0.750343166757458));
#5290=CARTESIAN_POINT('Ctrl Pts',(-21.4976674225048,-104.905021337286,-0.742238594469177));
#5291=CARTESIAN_POINT('Ctrl Pts',(-21.5466705229745,-104.676187630697,-0.742238594469178));
#5292=CARTESIAN_POINT('Ctrl Pts',(-21.5941724070256,-104.558712433615,-0.75034316675746));
#5293=CARTESIAN_POINT('Ctrl Pts',(-21.7287811554342,-104.351555835029,-0.782691551146546));
#5294=CARTESIAN_POINT('Ctrl Pts',(-21.8158438636493,-104.261835149209,-0.806867470269865));
#5295=CARTESIAN_POINT('Ctrl Pts',(-22.0050091877668,-104.122719505682,-0.862777168957507));
#5296=CARTESIAN_POINT('Ctrl Pts',(-22.1218994092456,-104.065586327466,-0.899065813509786));
#5297=CARTESIAN_POINT('Ctrl Pts',(-22.3070770846659,-104.016655879379,-0.958396191034765));
#5298=CARTESIAN_POINT('Ctrl Pts',(-22.3711029895888,-104.006315518874,-0.979199451876272));
#5299=CARTESIAN_POINT('Ctrl Pts',(-22.4343957334051,-104.002154280361,-1.00000000000001));
#5300=CARTESIAN_POINT('Origin',(-22.5,-100.,-1.50000000000001));
#5301=CARTESIAN_POINT('',(-22.5,-99.0000000000013,-1.00000000000001));
#5302=CARTESIAN_POINT('',(-22.5,-100.999999999999,-1.00000000000001));
#5303=CARTESIAN_POINT('Origin',(-22.4999999999999,-100.,-1.00000000000005));
#5304=CARTESIAN_POINT('Origin',(-22.4999999999992,-99.9999999999994,-0.999999999999742));
#5305=CARTESIAN_POINT('Origin',(-22.5,-95.0000000000001,-1.50000000000001));
#5306=CARTESIAN_POINT('',(-22.5,-94.0000000000013,-1.00000000000001));
#5307=CARTESIAN_POINT('',(-22.5,-95.9999999999988,-1.00000000000001));
#5308=CARTESIAN_POINT('Origin',(-22.5000000000019,-95.000000000002,-0.999999999999375));
#5309=CARTESIAN_POINT('Origin',(-22.4999999999992,-94.9999999999993,-0.999999999999733));
#5310=CARTESIAN_POINT('Origin',(-22.5,-90.0000000000001,-1.50000000000001));
#5311=CARTESIAN_POINT('',(-22.5,-89.0000000000013,-1.00000000000001));
#5312=CARTESIAN_POINT('',(-22.5,-90.9999999999988,-1.00000000000001));
#5313=CARTESIAN_POINT('Origin',(-22.5000000000003,-90.0000000000003,-0.999999999999934));
#5314=CARTESIAN_POINT('Origin',(-22.5000000000004,-90.0000000000005,-1.00000000000014));
#5315=CARTESIAN_POINT('Origin',(-22.5,-85.0000000000001,-1.50000000000001));
#5316=CARTESIAN_POINT('',(-22.5,-84.0000000000013,-1.00000000000001));
#5317=CARTESIAN_POINT('',(-22.5,-85.9999999999988,-1.00000000000001));
#5318=CARTESIAN_POINT('Origin',(-22.4999999999998,-85.,-1.00000000000009));
#5319=CARTESIAN_POINT('Origin',(-22.4999999999998,-84.9999999999999,-0.999999999999931));
#5320=CARTESIAN_POINT('Origin',(-22.5,-80.0000000000001,-1.50000000000001));
#5321=CARTESIAN_POINT('',(-22.4500000000001,-79.0012507822294,-1.00000000000001));
#5322=CARTESIAN_POINT('',(-21.5000000000012,-80.,-1.33333333333294));
#5323=CARTESIAN_POINT('Ctrl Pts',(-22.4500000000001,-79.0012507822294,-0.999999999999996));
#5324=CARTESIAN_POINT('Ctrl Pts',(-22.433178965212,-79.0020928872588,-1.00560701159605));
#5325=CARTESIAN_POINT('Ctrl Pts',(-22.4164991934282,-79.003354331563,-1.01118110520576));
#5326=CARTESIAN_POINT('Ctrl Pts',(-22.4000000000002,-79.0050125628946,-1.01670854297789));
#5327=CARTESIAN_POINT('Ctrl Pts',(-22.2827867384775,-79.0167929389226,-1.05597646307129));
#5328=CARTESIAN_POINT('Ctrl Pts',(-22.1591192674472,-79.0513996254551,-1.0981750197407));
#5329=CARTESIAN_POINT('Ctrl Pts',(-21.9333812202348,-79.1663420781321,-1.17665640788624));
#5330=CARTESIAN_POINT('Ctrl Pts',(-21.8313133719646,-79.2467073428857,-1.21290387580589));
#5331=CARTESIAN_POINT('Ctrl Pts',(-21.6759155424808,-79.4222458403709,-1.26875239207065));
#5332=CARTESIAN_POINT('Ctrl Pts',(-21.6097645938577,-79.5280963986251,-1.29290860193093));
#5333=CARTESIAN_POINT('Ctrl Pts',(-21.5217810563411,-79.7585465079784,-1.32523367161175));
#5334=CARTESIAN_POINT('Ctrl Pts',(-21.5000000000012,-79.8831754310448,-1.33333333333292));
#5335=CARTESIAN_POINT('Ctrl Pts',(-21.5000000000012,-80.0000000000001,-1.33333333333292));
#5336=CARTESIAN_POINT('',(-22.5,-80.9999999999988,-1.00000000000001));
#5337=CARTESIAN_POINT('Origin',(-22.4999999999997,-80.0000000000004,-1.00000000000013));
#5338=CARTESIAN_POINT('',(-21.5000000000012,-80.,-0.666666666667091));
#5339=CARTESIAN_POINT('Origin',(-22.4999999999995,-80.0000000000006,-0.999999999999846));
#5340=CARTESIAN_POINT('Ctrl Pts',(-21.5000000000012,-80.0000000000001,-0.666666666667071));
#5341=CARTESIAN_POINT('Ctrl Pts',(-21.5000000000012,-79.8831754310448,-0.666666666667072));
#5342=CARTESIAN_POINT('Ctrl Pts',(-21.5217810563411,-79.7585465079784,-0.67476632838824));
#5343=CARTESIAN_POINT('Ctrl Pts',(-21.6097645938577,-79.5280963986251,-0.707091398069062));
#5344=CARTESIAN_POINT('Ctrl Pts',(-21.6759155424808,-79.4222458403709,-0.731247607929342));
#5345=CARTESIAN_POINT('Ctrl Pts',(-21.8313133719646,-79.2467073428857,-0.787096124194101));
#5346=CARTESIAN_POINT('Ctrl Pts',(-21.9333812202348,-79.1663420781321,-0.823343592113753));
#5347=CARTESIAN_POINT('Ctrl Pts',(-22.1591192674472,-79.0513996254551,-0.901824980259289));
#5348=CARTESIAN_POINT('Ctrl Pts',(-22.2827867384775,-79.0167929389226,-0.944023536928704));
#5349=CARTESIAN_POINT('Ctrl Pts',(-22.4000000000002,-79.0050125628946,-0.983291457022097));
#5350=CARTESIAN_POINT('Ctrl Pts',(-22.4164991934282,-79.003354331563,-0.988818894794232));
#5351=CARTESIAN_POINT('Ctrl Pts',(-22.433178965212,-79.0020928872588,-0.994392988403943));
#5352=CARTESIAN_POINT('Ctrl Pts',(-22.4500000000001,-79.0012507822294,-0.999999999999997));
#5353=CARTESIAN_POINT('Origin',(-16.3268343236508,-70.7612046748876,-1.50000000000001));
#5354=CARTESIAN_POINT('',(-15.3849761916216,-70.4251938727838,-1.00000000000001));
#5355=CARTESIAN_POINT('',(-17.2304241124439,-71.1896034302417,-1.00000000000001));
#5356=CARTESIAN_POINT('Ctrl Pts',(-15.3849761916216,-70.4251938727838,-0.999999999999998));
#5357=CARTESIAN_POINT('Ctrl Pts',(-15.3793170638938,-70.4410567421835,-1.00560701159611));
#5358=CARTESIAN_POINT('Ctrl Pts',(-15.3740994141505,-70.4569495757777,-1.01118110520587));
#5359=CARTESIAN_POINT('Ctrl Pts',(-15.3693174521657,-70.4728274205466,-1.01670854297806));
#5360=CARTESIAN_POINT('Ctrl Pts',(-15.335345527225,-70.5856265085394,-1.0559764630715));
#5361=CARTESIAN_POINT('Ctrl Pts',(-15.3199924443146,-70.7131237594469,-1.09817501974097));
#5362=CARTESIAN_POINT('Ctrl Pts',(-15.3397992130368,-70.9656650932907,-1.17665640788659));
#5363=CARTESIAN_POINT('Ctrl Pts',(-15.3749873617574,-71.090717944594,-1.21290387580629));
#5364=CARTESIAN_POINT('Ctrl Pts',(-15.477695611983,-71.3014624933809,-1.26875239207111));
#5365=CARTESIAN_POINT('Ctrl Pts',(-15.5501739041858,-71.4030852558205,-1.29290860193142));
#5366=CARTESIAN_POINT('Ctrl Pts',(-15.729412201354,-71.5725608841664,-1.32523367161228));
#5367=CARTESIAN_POINT('Ctrl Pts',(-15.8362190631334,-71.6403773803664,-1.33333333333346));
#5368=CARTESIAN_POINT('Ctrl Pts',(-16.0520827194381,-71.7297910344313,-1.33333333333346));
#5369=CARTESIAN_POINT('Ctrl Pts',(-16.1755600800189,-71.7573613863334,-1.32523367161228));
#5370=CARTESIAN_POINT('Ctrl Pts',(-16.4221380614441,-71.7642646356601,-1.29290860193142));
#5371=CARTESIAN_POINT('Ctrl Pts',(-16.5452460977935,-71.7436563831215,-1.26875239207111));
#5372=CARTESIAN_POINT('Ctrl Pts',(-16.7668906975571,-71.6672631837946,-1.21290387580629));
#5373=CARTESIAN_POINT('Ctrl Pts',(-16.8801981952981,-71.6037192432091,-1.1766564078866));
#5374=CARTESIAN_POINT('Ctrl Pts',(-17.0727773854659,-71.4391510539951,-1.09817501974097));
#5375=CARTESIAN_POINT('Ctrl Pts',(-17.1520752871271,-71.3381406142577,-1.0559764630715));
#5376=CARTESIAN_POINT('Ctrl Pts',(-17.2156604826226,-71.2197491462776,-1.01118110520602));
#5377=CARTESIAN_POINT('Ctrl Pts',(-17.2232089775138,-71.204821780356,-1.0056070115964));
#5378=CARTESIAN_POINT('Ctrl Pts',(-17.2304241124433,-71.1896034302429,-1.00000000000044));
#5379=CARTESIAN_POINT('Ctrl Pts',(-17.2304241124439,-71.1896034302417,-1.));
#5380=CARTESIAN_POINT('Ctrl Pts',(-17.2232089775142,-71.2048217803552,-0.994392988403892));
#5381=CARTESIAN_POINT('Ctrl Pts',(-17.2156604826228,-71.2197491462772,-0.988818894794122));
#5382=CARTESIAN_POINT('Ctrl Pts',(-17.1520752871271,-71.3381406142577,-0.944023536928495));
#5383=CARTESIAN_POINT('Ctrl Pts',(-17.0727773854659,-71.4391510539951,-0.901824980259031));
#5384=CARTESIAN_POINT('Ctrl Pts',(-16.8801981952981,-71.6037192432091,-0.823343592113403));
#5385=CARTESIAN_POINT('Ctrl Pts',(-16.7668906975571,-71.6672631837946,-0.787096124193711));
#5386=CARTESIAN_POINT('Ctrl Pts',(-16.5452460977935,-71.7436563831215,-0.731247607928886));
#5387=CARTESIAN_POINT('Ctrl Pts',(-16.4221380614441,-71.7642646356601,-0.707091398068581));
#5388=CARTESIAN_POINT('Ctrl Pts',(-16.1755600800189,-71.7573613863334,-0.674766328387719));
#5389=CARTESIAN_POINT('Ctrl Pts',(-16.0520827194381,-71.7297910344313,-0.666666666666536));
#5390=CARTESIAN_POINT('Ctrl Pts',(-15.8362190631334,-71.6403773803664,-0.666666666666536));
#5391=CARTESIAN_POINT('Ctrl Pts',(-15.729412201354,-71.5725608841664,-0.674766328387716));
#5392=CARTESIAN_POINT('Ctrl Pts',(-15.5501739041858,-71.4030852558205,-0.707091398068578));
#5393=CARTESIAN_POINT('Ctrl Pts',(-15.477695611983,-71.3014624933809,-0.731247607928885));
#5394=CARTESIAN_POINT('Ctrl Pts',(-15.3749873617574,-71.090717944594,-0.78709612419371));
#5395=CARTESIAN_POINT('Ctrl Pts',(-15.3397992130368,-70.9656650932907,-0.823343592113405));
#5396=CARTESIAN_POINT('Ctrl Pts',(-15.3199924443146,-70.7131237594469,-0.901824980259028));
#5397=CARTESIAN_POINT('Ctrl Pts',(-15.335345527225,-70.5856265085394,-0.944023536928495));
#5398=CARTESIAN_POINT('Ctrl Pts',(-15.3693174521657,-70.4728274205466,-0.983291457021933));
#5399=CARTESIAN_POINT('Ctrl Pts',(-15.3740994141504,-70.4569495757781,-0.988818894793977));
#5400=CARTESIAN_POINT('Ctrl Pts',(-15.3793170638935,-70.4410567421843,-0.994392988403597));
#5401=CARTESIAN_POINT('Ctrl Pts',(-15.3849761916211,-70.4251938727851,-0.999999999999556));
#5402=CARTESIAN_POINT('Origin',(-19.5710678118652,-72.9289321881353,-1.50000000000001));
#5403=CARTESIAN_POINT('',(-18.8294901282151,-72.2580651826028,-1.00000000000001));
#5404=CARTESIAN_POINT('',(-20.2419348173977,-73.6705098717854,-1.00000000000001));
#5405=CARTESIAN_POINT('Ctrl Pts',(-18.8294901282151,-72.2580651826028,-0.999999999999999));
#5406=CARTESIAN_POINT('Ctrl Pts',(-18.8181913186264,-72.270554908545,-1.00560701159615));
#5407=CARTESIAN_POINT('Ctrl Pts',(-18.8072889147109,-72.2832412641038,-1.01118110520595));
#5408=CARTESIAN_POINT('Ctrl Pts',(-18.796794769773,-72.2960805022804,-1.01670854297818));
#5409=CARTESIAN_POINT('Ctrl Pts',(-18.7222424614796,-72.3872927781225,-1.05597646307161));
#5410=CARTESIAN_POINT('Ctrl Pts',(-18.6592669768233,-72.4992095082219,-1.09817501974108));
#5411=CARTESIAN_POINT('Ctrl Pts',(-18.5809226606016,-72.740106999912,-1.17665640788671));
#5412=CARTESIAN_POINT('Ctrl Pts',(-18.5655766166277,-72.8691066912443,-1.2129038758064));
#5413=CARTESIAN_POINT('Ctrl Pts',(-18.5798182195492,-73.1031140121853,-1.26875239207123));
#5414=CARTESIAN_POINT('Ctrl Pts',(-18.6078900827299,-73.2247374440727,-1.29290860193154));
#5415=CARTESIAN_POINT('Ctrl Pts',(-18.7086291617681,-73.4499040351326,-1.3252336716124));
#5416=CARTESIAN_POINT('Ctrl Pts',(-18.7813535857611,-73.5534315244043,-1.33333333333357));
#5417=CARTESIAN_POINT('Ctrl Pts',(-18.9465684755962,-73.7186464142394,-1.33333333333357));
#5418=CARTESIAN_POINT('Ctrl Pts',(-19.0500959648678,-73.7913708382324,-1.32523367161239));
#5419=CARTESIAN_POINT('Ctrl Pts',(-19.2752625559277,-73.8921099172706,-1.29290860193153));
#5420=CARTESIAN_POINT('Ctrl Pts',(-19.3968859878151,-73.9201817804513,-1.26875239207122));
#5421=CARTESIAN_POINT('Ctrl Pts',(-19.6308933087562,-73.9344233833728,-1.2129038758064));
#5422=CARTESIAN_POINT('Ctrl Pts',(-19.7598930000884,-73.9190773393989,-1.17665640788671));
#5423=CARTESIAN_POINT('Ctrl Pts',(-20.0007904917785,-73.8407330231772,-1.09817501974108));
#5424=CARTESIAN_POINT('Ctrl Pts',(-20.1127072218779,-73.7777575385209,-1.05597646307161));
#5425=CARTESIAN_POINT('Ctrl Pts',(-20.2167587358963,-73.6927110852899,-1.01118110520609));
#5426=CARTESIAN_POINT('Ctrl Pts',(-20.2294450914547,-73.6818086813747,-1.00560701159644));
#5427=CARTESIAN_POINT('Ctrl Pts',(-20.2419348173967,-73.6705098717863,-1.00000000000044));
#5428=CARTESIAN_POINT('Ctrl Pts',(-20.2419348173977,-73.6705098717854,-0.999999999999999));
#5429=CARTESIAN_POINT('Ctrl Pts',(-20.2294450914554,-73.6818086813741,-0.994392988403851));
#5430=CARTESIAN_POINT('Ctrl Pts',(-20.2167587358967,-73.6927110852896,-0.988818894794047));
#5431=CARTESIAN_POINT('Ctrl Pts',(-20.1127072218779,-73.7777575385209,-0.944023536928382));
#5432=CARTESIAN_POINT('Ctrl Pts',(-20.0007904917785,-73.8407330231772,-0.901824980258916));
#5433=CARTESIAN_POINT('Ctrl Pts',(-19.7598930000884,-73.9190773393989,-0.823343592113289));
#5434=CARTESIAN_POINT('Ctrl Pts',(-19.6308933087562,-73.9344233833728,-0.787096124193595));
#5435=CARTESIAN_POINT('Ctrl Pts',(-19.3968859878151,-73.9201817804513,-0.73124760792877));
#5436=CARTESIAN_POINT('Ctrl Pts',(-19.2752625559277,-73.8921099172706,-0.707091398068464));
#5437=CARTESIAN_POINT('Ctrl Pts',(-19.0500959648678,-73.7913708382324,-0.674766328387601));
#5438=CARTESIAN_POINT('Ctrl Pts',(-18.9465684755962,-73.7186464142394,-0.666666666666421));
#5439=CARTESIAN_POINT('Ctrl Pts',(-18.7813535857611,-73.5534315244043,-0.666666666666421));
#5440=CARTESIAN_POINT('Ctrl Pts',(-18.7086291617681,-73.4499040351326,-0.674766328387602));
#5441=CARTESIAN_POINT('Ctrl Pts',(-18.6078900827299,-73.2247374440727,-0.707091398068464));
#5442=CARTESIAN_POINT('Ctrl Pts',(-18.5798182195492,-73.1031140121853,-0.731247607928769));
#5443=CARTESIAN_POINT('Ctrl Pts',(-18.5655766166277,-72.8691066912443,-0.787096124193594));
#5444=CARTESIAN_POINT('Ctrl Pts',(-18.5809226606016,-72.740106999912,-0.823343592113288));
#5445=CARTESIAN_POINT('Ctrl Pts',(-18.6592669768233,-72.4992095082219,-0.901824980258915));
#5446=CARTESIAN_POINT('Ctrl Pts',(-18.7222424614796,-72.3872927781225,-0.944023536928382));
#5447=CARTESIAN_POINT('Ctrl Pts',(-18.796794769773,-72.2960805022804,-0.98329145702182));
#5448=CARTESIAN_POINT('Ctrl Pts',(-18.8072889147106,-72.2832412641041,-0.9888188947939));
#5449=CARTESIAN_POINT('Ctrl Pts',(-18.8181913186258,-72.2705549085457,-0.994392988403553));
#5450=CARTESIAN_POINT('Ctrl Pts',(-18.8294901282142,-72.2580651826038,-0.99999999999955));
#5451=CARTESIAN_POINT('Origin',(-21.7387953251129,-76.1731656763492,-1.50000000000001));
#5452=CARTESIAN_POINT('',(-21.3103965697588,-75.269575887557,-1.00000000000001));
#5453=CARTESIAN_POINT('',(-22.074806127216,-77.1150238083777,-1.00000000000001));
#5454=CARTESIAN_POINT('Ctrl Pts',(-21.3103965697588,-75.269575887557,-1.));
#5455=CARTESIAN_POINT('Ctrl Pts',(-21.2951782196454,-75.2767910224866,-1.00560701159606));
#5456=CARTESIAN_POINT('Ctrl Pts',(-21.2802508537235,-75.2843395173779,-1.01118110520577));
#5457=CARTESIAN_POINT('Ctrl Pts',(-21.2656421642701,-75.2921854913377,-1.01670854297791));
#5458=CARTESIAN_POINT('Ctrl Pts',(-21.1618593857433,-75.3479247128735,-1.05597646307131));
#5459=CARTESIAN_POINT('Ctrl Pts',(-21.060848946006,-75.4272226145347,-1.09817501974074));
#5460=CARTESIAN_POINT('Ctrl Pts',(-20.8962807567921,-75.6198018047023,-1.17665640788631));
#5461=CARTESIAN_POINT('Ctrl Pts',(-20.8327368162066,-75.7331093024432,-1.21290387580597));
#5462=CARTESIAN_POINT('Ctrl Pts',(-20.7563436168797,-75.9547539022067,-1.26875239207076));
#5463=CARTESIAN_POINT('Ctrl Pts',(-20.7357353643411,-76.077861938556,-1.29290860193104));
#5464=CARTESIAN_POINT('Ctrl Pts',(-20.7426386136678,-76.324439919981,-1.32523367161188));
#5465=CARTESIAN_POINT('Ctrl Pts',(-20.77020896557,-76.4479172805617,-1.33333333333305));
#5466=CARTESIAN_POINT('Ctrl Pts',(-20.8596226196347,-76.6637809368662,-1.33333333333305));
#5467=CARTESIAN_POINT('Ctrl Pts',(-20.9274391158347,-76.7705877986455,-1.32523367161188));
#5468=CARTESIAN_POINT('Ctrl Pts',(-21.0969147441805,-76.9498260958136,-1.29290860193104));
#5469=CARTESIAN_POINT('Ctrl Pts',(-21.1985375066201,-77.0223043880163,-1.26875239207076));
#5470=CARTESIAN_POINT('Ctrl Pts',(-21.4092820554068,-77.1250126382418,-1.21290387580597));
#5471=CARTESIAN_POINT('Ctrl Pts',(-21.5343349067099,-77.1602007869623,-1.17665640788631));
#5472=CARTESIAN_POINT('Ctrl Pts',(-21.7868762405536,-77.1800075556846,-1.09817501974075));
#5473=CARTESIAN_POINT('Ctrl Pts',(-21.914373491461,-77.1646544727742,-1.05597646307131));
#5474=CARTESIAN_POINT('Ctrl Pts',(-22.043050424222,-77.1259005858488,-1.01118110520591));
#5475=CARTESIAN_POINT('Ctrl Pts',(-22.0589432578156,-77.1206829361058,-1.00560701159635));
#5476=CARTESIAN_POINT('Ctrl Pts',(-22.0748061272147,-77.1150238083782,-1.00000000000044));
#5477=CARTESIAN_POINT('Ctrl Pts',(-22.074806127216,-77.1150238083777,-0.999999999999997));
#5478=CARTESIAN_POINT('Ctrl Pts',(-22.0589432578165,-77.1206829361055,-0.994392988403939));
#5479=CARTESIAN_POINT('Ctrl Pts',(-22.0430504242224,-77.1259005858487,-0.988818894794226));
#5480=CARTESIAN_POINT('Ctrl Pts',(-21.914373491461,-77.1646544727742,-0.94402353692868));
#5481=CARTESIAN_POINT('Ctrl Pts',(-21.7868762405536,-77.1800075556846,-0.901824980259249));
#5482=CARTESIAN_POINT('Ctrl Pts',(-21.5343349067099,-77.1602007869623,-0.823343592113684));
#5483=CARTESIAN_POINT('Ctrl Pts',(-21.4092820554068,-77.1250126382418,-0.787096124194018));
#5484=CARTESIAN_POINT('Ctrl Pts',(-21.1985375066201,-77.0223043880163,-0.731247607929237));
#5485=CARTESIAN_POINT('Ctrl Pts',(-21.0969147441805,-76.9498260958136,-0.707091398068949));
#5486=CARTESIAN_POINT('Ctrl Pts',(-20.9274391158347,-76.7705877986455,-0.674766328388114));
#5487=CARTESIAN_POINT('Ctrl Pts',(-20.8596226196347,-76.6637809368662,-0.66666666666694));
#5488=CARTESIAN_POINT('Ctrl Pts',(-20.77020896557,-76.4479172805617,-0.66666666666694));
#5489=CARTESIAN_POINT('Ctrl Pts',(-20.7426386136678,-76.324439919981,-0.674766328388116));
#5490=CARTESIAN_POINT('Ctrl Pts',(-20.7357353643411,-76.0778619385559,-0.707091398068951));
#5491=CARTESIAN_POINT('Ctrl Pts',(-20.7563436168797,-75.9547539022067,-0.731247607929234));
#5492=CARTESIAN_POINT('Ctrl Pts',(-20.8327368162066,-75.7331093024432,-0.787096124194015));
#5493=CARTESIAN_POINT('Ctrl Pts',(-20.8962807567921,-75.6198018047023,-0.823343592113683));
#5494=CARTESIAN_POINT('Ctrl Pts',(-21.060848946006,-75.4272226145347,-0.901824980259247));
#5495=CARTESIAN_POINT('Ctrl Pts',(-21.1618593857433,-75.3479247128735,-0.944023536928678));
#5496=CARTESIAN_POINT('Ctrl Pts',(-21.2656421642701,-75.2921854913377,-0.983291457022086));
#5497=CARTESIAN_POINT('Ctrl Pts',(-21.2802508537231,-75.2843395173782,-0.988818894794077));
#5498=CARTESIAN_POINT('Ctrl Pts',(-21.2951782196446,-75.276791022487,-0.994392988403642));
#5499=CARTESIAN_POINT('Ctrl Pts',(-21.3103965697576,-75.2695758875576,-0.999999999999549));
#5500=CARTESIAN_POINT('Origin',(-19.5,-120.,-2.00000000000001));
#5501=CARTESIAN_POINT('',(-19.5,-116.5,-2.00000000000001));
#5502=CARTESIAN_POINT('',(-19.5,-102.858571571457,-2.00000000000001));
#5503=CARTESIAN_POINT('',(-19.5,-120.,-2.00000000000001));
#5504=CARTESIAN_POINT('',(-19.5,-116.5,-1.38777878078145E-14));
#5505=CARTESIAN_POINT('',(-19.5,-116.5,-2.00000000000001));
#5506=CARTESIAN_POINT('',(-19.5,-102.858571571457,-1.38777878078145E-14));
#5507=CARTESIAN_POINT('',(-19.5,-120.,-1.38777878078145E-14));
#5508=CARTESIAN_POINT('',(-19.5,-110.,-1.00000000000001));
#5509=CARTESIAN_POINT('Ctrl Pts',(-19.5,-102.858571571457,-1.91247983633255E-14));
#5510=CARTESIAN_POINT('Ctrl Pts',(-19.5,-105.799159747916,-2.57409313859276E-14));
#5511=CARTESIAN_POINT('Ctrl Pts',(-19.5,-110.,-0.999999999999999));
#5512=CARTESIAN_POINT('Ctrl Pts',(-19.5,-110.,-0.999999999999988));
#5513=CARTESIAN_POINT('Ctrl Pts',(-19.5,-105.799159747916,-2.));
#5514=CARTESIAN_POINT('Ctrl Pts',(-19.5,-102.858571571457,-2.));
#5515=CARTESIAN_POINT('Origin',(-12.5,-120.,-2.00000000000001));
#5516=CARTESIAN_POINT('',(-12.5,-116.5,-1.38777878078145E-14));
#5517=CARTESIAN_POINT('',(-12.5,-73.0000000000001,0.));
#5518=CARTESIAN_POINT('',(-12.5,-120.,-1.38777878078145E-14));
#5519=CARTESIAN_POINT('',(-12.5,-116.5,-2.00000000000001));
#5520=CARTESIAN_POINT('',(-12.5,-116.5,-2.00000000000001));
#5521=CARTESIAN_POINT('',(-12.5,-73.0000000000001,-2.));
#5522=CARTESIAN_POINT('',(-12.5,-120.,-2.00000000000001));
#5523=CARTESIAN_POINT('',(-12.5,-71.0000000000001,-1.33333333333334));
#5524=CARTESIAN_POINT('',(-12.5,-80.,-4.3333333333333));
#5525=CARTESIAN_POINT('',(-12.5,-71.0000000000001,-0.66666666666667));
#5526=CARTESIAN_POINT('',(-12.5,-71.0000000000001,-1.50000000000001));
#5527=CARTESIAN_POINT('',(-12.5,-80.,2.3333333333333));
#5528=CARTESIAN_POINT('Origin',(0.,-5.55111146474324E-17,-2.));
#5529=CARTESIAN_POINT('Origin',(-16.,-116.5,-2.00000000000001));
#5530=CARTESIAN_POINT('',(-19.5,-80.,-2.00000000000001));
#5531=CARTESIAN_POINT('',(-19.5,-1.40859542590934E-15,-2.00000000000001));
#5532=CARTESIAN_POINT('Origin',(-12.5,-80.,-2.));
#5533=CARTESIAN_POINT('Origin',(0.,0.,0.));
#5534=CARTESIAN_POINT('Origin',(-16.,-116.5,-1.38777878078145E-14));
#5535=CARTESIAN_POINT('',(-19.5,-80.,-1.38777878078145E-14));
#5536=CARTESIAN_POINT('Origin',(-12.5,-80.,0.));
#5537=CARTESIAN_POINT('',(-19.5,-102.858571571457,-1.38777878078145E-14));
#5538=CARTESIAN_POINT('Origin',(-12.5,-102.858571571457,-1.38777878078145E-14));
#5539=CARTESIAN_POINT('Origin',(-12.5,-102.858571571457,-1.00000000000001));
#5540=CARTESIAN_POINT('',(-22.5,-102.858571571457,-1.00000000000001));
#5541=CARTESIAN_POINT('',(-22.5,-102.858571571457,-1.00000000000001));
#5542=CARTESIAN_POINT('Origin',(-12.5,-102.858571571457,-1.00000000000001));
#5543=CARTESIAN_POINT('Origin',(-22.5,-1.58900668570284E-15,-1.00000000000001));
#5544=CARTESIAN_POINT('',(-22.5,-80.,-1.00000000000001));
#5545=CARTESIAN_POINT('',(-22.5,-80.,-1.00000000000001));
#5546=CARTESIAN_POINT('',(-22.5,-80.,-1.00000000000001));
#5547=CARTESIAN_POINT('',(-22.5,-80.,-1.00000000000001));
#5548=CARTESIAN_POINT('',(-22.5,-80.,-1.00000000000001));
#5549=CARTESIAN_POINT('',(-22.5,-80.,-1.00000000000001));
#5550=CARTESIAN_POINT('Origin',(-12.5,-102.858571571457,-2.00000000000001));
#5551=CARTESIAN_POINT('',(-19.5,-102.858571571457,-2.00000000000001));
#5552=CARTESIAN_POINT('Origin',(-12.5,-80.,0.));
#5553=CARTESIAN_POINT('',(-13.4987492177719,-70.05,-1.00000000000001));
#5554=CARTESIAN_POINT('Ctrl Pts',(-13.4987492177719,-70.05,-1.));
#5555=CARTESIAN_POINT('Ctrl Pts',(-13.4979071127425,-70.0668210347882,-0.994392988403934));
#5556=CARTESIAN_POINT('Ctrl Pts',(-13.4966456684383,-70.083500806572,-0.988818894794213));
#5557=CARTESIAN_POINT('Ctrl Pts',(-13.4832070610786,-70.2172132615229,-0.944023536928626));
#5558=CARTESIAN_POINT('Ctrl Pts',(-13.4486003745461,-70.3408807325533,-0.90182498025916));
#5559=CARTESIAN_POINT('Ctrl Pts',(-13.333657921869,-70.5666187797661,-0.823343592113535));
#5560=CARTESIAN_POINT('Ctrl Pts',(-13.2532926571153,-70.6686866280364,-0.78709612419384));
#5561=CARTESIAN_POINT('Ctrl Pts',(-13.0777541596298,-70.8240844575203,-0.731247607929015));
#5562=CARTESIAN_POINT('Ctrl Pts',(-12.9719036013755,-70.8902354061435,-0.707091398068708));
#5563=CARTESIAN_POINT('Ctrl Pts',(-12.7414534920219,-70.9782189436602,-0.674766328387846));
#5564=CARTESIAN_POINT('Ctrl Pts',(-12.6168245689554,-71.0000000000001,-0.666666666666663));
#5565=CARTESIAN_POINT('Ctrl Pts',(-12.5,-71.0000000000001,-0.666666666666664));
#5566=CARTESIAN_POINT('Origin',(-12.5,-80.,-1.00000000000001));
#5567=CARTESIAN_POINT('Origin',(-12.5,-80.,-1.00000000000001));
#5568=CARTESIAN_POINT('Origin',(-12.5,-80.,-1.00000000000001));
#5569=CARTESIAN_POINT('Origin',(-12.5,-80.,-1.00000000000001));
#5570=CARTESIAN_POINT('Origin',(-22.5,-1.58900668570284E-15,-1.00000000000001));
#5571=CARTESIAN_POINT('',(-19.5,-80.,-2.00000000000001));
#5572=CARTESIAN_POINT('Origin',(-12.5,-80.,-2.));
#5573=CARTESIAN_POINT('Ctrl Pts',(-12.5,-71.0000000000001,-1.33333333333334));
#5574=CARTESIAN_POINT('Ctrl Pts',(-12.6168245689554,-71.0000000000001,-1.33333333333334));
#5575=CARTESIAN_POINT('Ctrl Pts',(-12.7414534920219,-70.9782189436602,-1.32523367161216));
#5576=CARTESIAN_POINT('Ctrl Pts',(-12.9719036013755,-70.8902354061435,-1.29290860193129));
#5577=CARTESIAN_POINT('Ctrl Pts',(-13.0777541596298,-70.8240844575203,-1.26875239207099));
#5578=CARTESIAN_POINT('Ctrl Pts',(-13.2532926571153,-70.6686866280364,-1.21290387580616));
#5579=CARTESIAN_POINT('Ctrl Pts',(-13.333657921869,-70.5666187797661,-1.17665640788646));
#5580=CARTESIAN_POINT('Ctrl Pts',(-13.4486003745461,-70.3408807325533,-1.09817501974084));
#5581=CARTESIAN_POINT('Ctrl Pts',(-13.4832070610786,-70.2172132615229,-1.05597646307137));
#5582=CARTESIAN_POINT('Ctrl Pts',(-13.4966456684383,-70.083500806572,-1.01118110520579));
#5583=CARTESIAN_POINT('Ctrl Pts',(-13.4979071127425,-70.0668210347882,-1.00560701159606));
#5584=CARTESIAN_POINT('Ctrl Pts',(-13.4987492177719,-70.05,-0.999999999999998));
#5585=CARTESIAN_POINT('Origin',(-12.5,-70.,-1.50000000000001));
#5586=CARTESIAN_POINT('Origin',(-16.,-116.5,-2.00000000000001));
#5977=UNCERTAINTY_MEASURE_WITH_UNIT(LENGTH_MEASURE(0.01),#5991,
'DISTANCE_ACCURACY_VALUE',
'Maximum model space distance between geometric entities at asserted c
onnectivities');
#5981=UNCERTAINTY_MEASURE_WITH_UNIT(LENGTH_MEASURE(0.01),#5991,
'DISTANCE_ACCURACY_VALUE',
'Maximum model space distance between geometric entities at asserted c
onnectivities');
#5986=(
GEOMETRIC_REPRESENTATION_CONTEXT(3)
GLOBAL_UNCERTAINTY_ASSIGNED_CONTEXT((#5977))
GLOBAL_UNIT_ASSIGNED_CONTEXT((#5991,#5993,#5994))
REPRESENTATION_CONTEXT('','3D')
);
#5990=(
GEOMETRIC_REPRESENTATION_CONTEXT(3)
GLOBAL_UNCERTAINTY_ASSIGNED_CONTEXT((#5981))
GLOBAL_UNIT_ASSIGNED_CONTEXT((#5991,#5993,#5994))
REPRESENTATION_CONTEXT('','3D')
);
#5991=(
LENGTH_UNIT()
NAMED_UNIT(*)
SI_UNIT(.MILLI.,.METRE.)
);
#5993=(
NAMED_UNIT(*)
PLANE_ANGLE_UNIT()
SI_UNIT($,.RADIAN.)
);
#5994=(
NAMED_UNIT(*)
SI_UNIT($,.STERADIAN.)
SOLID_ANGLE_UNIT()
);
#5999=SHAPE_DEFINITION_REPRESENTATION(#6007,#6024);
#6007=PRODUCT_DEFINITION_SHAPE('',$,#6033);
#6024=SHAPE_REPRESENTATION('',(#3540),#5986);
#6028=PRODUCT_DEFINITION_CONTEXT('part definition',#6054,'design');
#6033=PRODUCT_DEFINITION('serrated knife','serrated knife',#6041,#6028);
#6041=PRODUCT_DEFINITION_FORMATION('',$,#6060);
#6054=APPLICATION_CONTEXT(
'Core Data for Automotive Mechanical Design Process');
#6055=PRODUCT_CONTEXT('part definition',#6054,'mechanical');
#6060=PRODUCT('serrated knife','serrated knife',$,(#6055));
#6066=PRESENTATION_STYLE_ASSIGNMENT((#6072));
#6072=SURFACE_STYLE_USAGE(.BOTH.,#6078);
#6078=SURFACE_SIDE_STYLE('',(#6084));
#6084=SURFACE_STYLE_FILL_AREA(#6090);
#6090=FILL_AREA_STYLE('Opaque(97,158,199)',(#6096));
#6096=FILL_AREA_STYLE_COLOUR('Opaque(97,158,199)',#6102);
#6102=COLOUR_RGB('Opaque(97,158,199)',0.380392156862745,0.619607843137255,
0.780392156862745);
ENDSEC;
END-ISO-10303-21;
